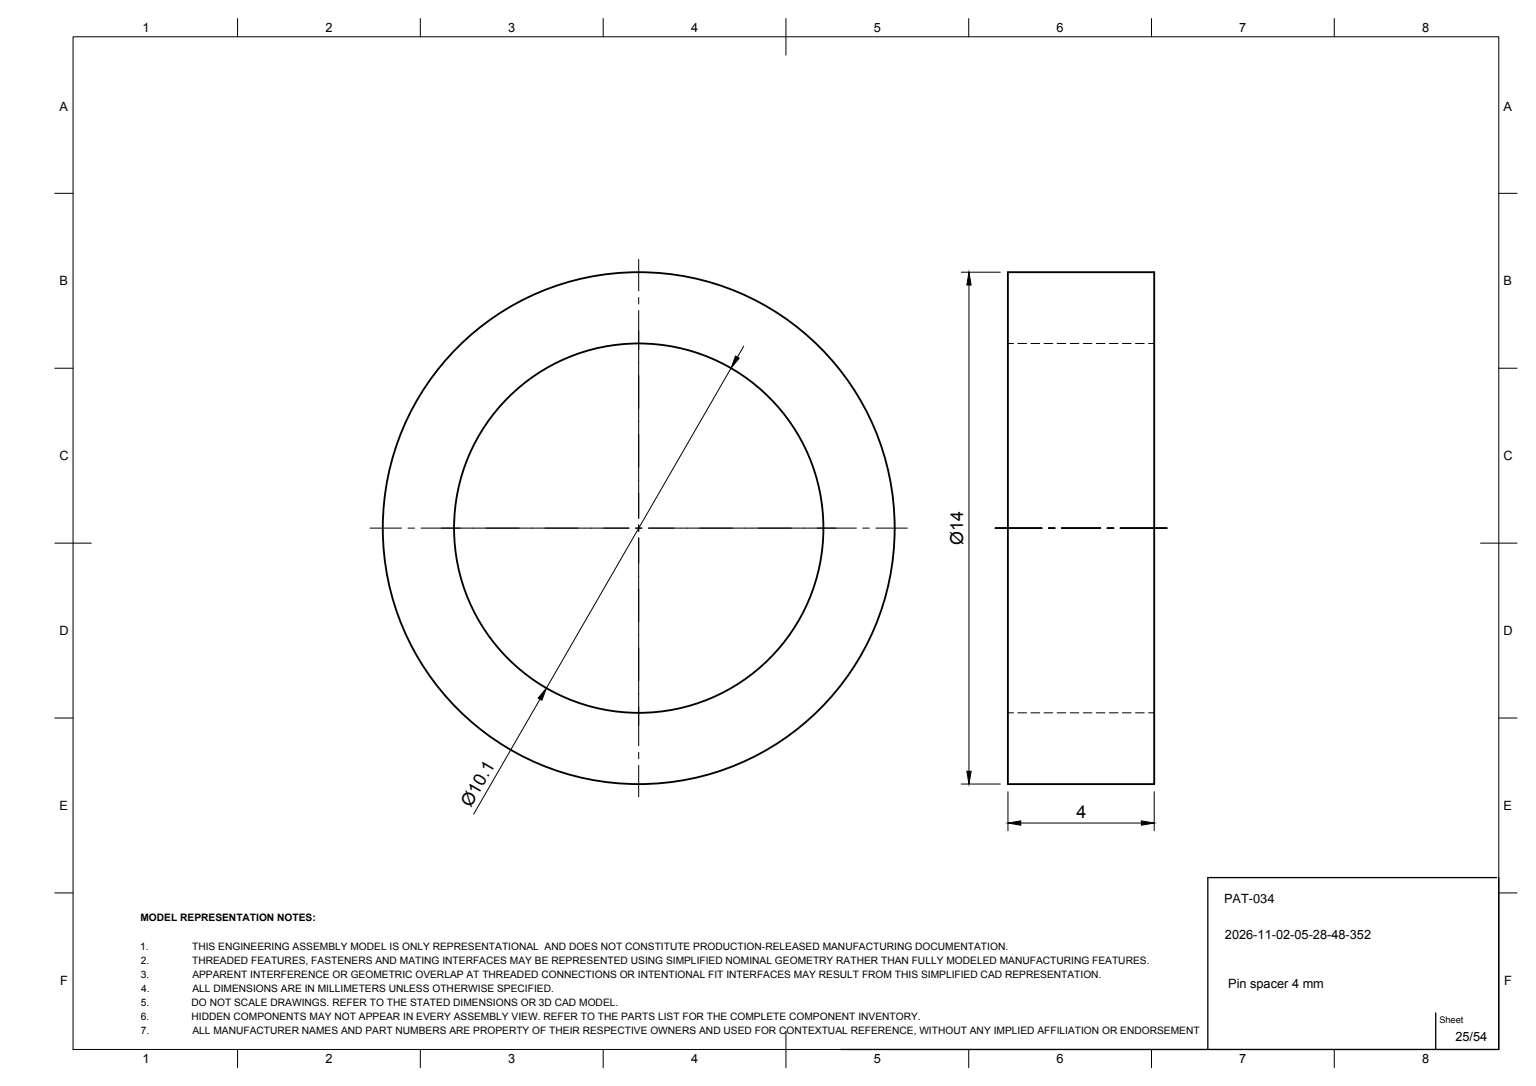
ISO-10303-21;
HEADER;
/* Generated by software containing ST-Developer
 * from STEP Tools, Inc. (www.steptools.com) 
 */

FILE_DESCRIPTION(
/* description */ ('Fatigue rig crank-slider'),
/* implementation_level */ '2;1');

FILE_NAME(
/* name */ 'Pin spacer 4 mm.step',
/* time_stamp */ '2026-10-28T03:24:50-07:00',
/* author */ (''),
/* organization */ (''),
/* preprocessor_version */ 'ST-DEVELOPER v20.2',
/* originating_system */ 'Autodesk Translation Framework v15.17.0.0',
/* authorisation */ '');

FILE_SCHEMA (('AUTOMOTIVE_DESIGN { 1 0 10303 214 3 1 1 }'));
ENDSEC;

DATA;
#10=MECHANICAL_DESIGN_GEOMETRIC_PRESENTATION_REPRESENTATION('',(#611),#16911);
#510=SHAPE_REPRESENTATION_RELATIONSHIP('SRR','None',#17151,#560);
#560=ADVANCED_BREP_SHAPE_REPRESENTATION('',(#668),#16880);
#611=STYLED_ITEM('',(#17487),#668);
#668=MANIFOLD_SOLID_BREP('Body1',#8904);
#837=FACE_BOUND('',#2151,.T.);
#838=FACE_BOUND('',#2153,.T.);
#1059=PLANE('',#10013);
#1060=PLANE('',#10014);
#1488=FACE_OUTER_BOUND('',#2148,.T.);
#1489=FACE_OUTER_BOUND('',#2149,.T.);
#1490=FACE_OUTER_BOUND('',#2150,.T.);
#1491=FACE_OUTER_BOUND('',#2152,.T.);
#2148=EDGE_LOOP('',(#7134,#7135,#7136,#7137));
#2149=EDGE_LOOP('',(#7138,#7139,#7140,#7141));
#2150=EDGE_LOOP('',(#7142));
#2151=EDGE_LOOP('',(#7143));
#2152=EDGE_LOOP('',(#7144));
#2153=EDGE_LOOP('',(#7145));
#2780=LINE('',#15198,#3426);
#2781=LINE('',#15204,#3427);
#3426=VECTOR('',#11918,0.505);
#3427=VECTOR('',#11925,0.7);
#3965=CIRCLE('',#10008,0.505);
#3966=CIRCLE('',#10009,0.505);
#3967=CIRCLE('',#10011,0.7);
#3968=CIRCLE('',#10012,0.7);
#4537=VERTEX_POINT('',#15195);
#4538=VERTEX_POINT('',#15197);
#4539=VERTEX_POINT('',#15201);
#4540=VERTEX_POINT('',#15203);
#5465=EDGE_CURVE('',#4537,#4537,#3965,.T.);
#5466=EDGE_CURVE('',#4537,#4538,#2780,.T.);
#5467=EDGE_CURVE('',#4538,#4538,#3966,.T.);
#5468=EDGE_CURVE('',#4539,#4539,#3967,.T.);
#5469=EDGE_CURVE('',#4539,#4540,#2781,.T.);
#5470=EDGE_CURVE('',#4540,#4540,#3968,.T.);
#7134=ORIENTED_EDGE('',*,*,#5465,.F.);
#7135=ORIENTED_EDGE('',*,*,#5466,.T.);
#7136=ORIENTED_EDGE('',*,*,#5467,.T.);
#7137=ORIENTED_EDGE('',*,*,#5466,.F.);
#7138=ORIENTED_EDGE('',*,*,#5468,.F.);
#7139=ORIENTED_EDGE('',*,*,#5469,.T.);
#7140=ORIENTED_EDGE('',*,*,#5470,.T.);
#7141=ORIENTED_EDGE('',*,*,#5469,.F.);
#7142=ORIENTED_EDGE('',*,*,#5468,.T.);
#7143=ORIENTED_EDGE('',*,*,#5465,.T.);
#7144=ORIENTED_EDGE('',*,*,#5470,.F.);
#7145=ORIENTED_EDGE('',*,*,#5467,.F.);
#8296=CYLINDRICAL_SURFACE('',#10007,0.505);
#8297=CYLINDRICAL_SURFACE('',#10010,0.7);
#8626=ADVANCED_FACE('',(#1488),#8296,.F.);
#8627=ADVANCED_FACE('',(#1489),#8297,.T.);
#8628=ADVANCED_FACE('',(#1490,#837),#1059,.T.);
#8629=ADVANCED_FACE('',(#1491,#838),#1060,.F.);
#8904=CLOSED_SHELL('',(#8626,#8627,#8628,#8629));
#10006=AXIS2_PLACEMENT_3D('',#15193,#11912,#11913);
#10007=AXIS2_PLACEMENT_3D('',#15194,#11914,#11915);
#10008=AXIS2_PLACEMENT_3D('',#15196,#11916,#11917);
#10009=AXIS2_PLACEMENT_3D('',#15199,#11919,#11920);
#10010=AXIS2_PLACEMENT_3D('',#15200,#11921,#11922);
#10011=AXIS2_PLACEMENT_3D('',#15202,#11923,#11924);
#10012=AXIS2_PLACEMENT_3D('',#15205,#11926,#11927);
#10013=AXIS2_PLACEMENT_3D('',#15206,#11928,#11929);
#10014=AXIS2_PLACEMENT_3D('',#15207,#11930,#11931);
#11912=DIRECTION('axis',(0.,0.,1.));
#11913=DIRECTION('refdir',(1.,0.,0.));
#11914=DIRECTION('center_axis',(0.,1.,0.));
#11915=DIRECTION('ref_axis',(1.,0.,0.));
#11916=DIRECTION('center_axis',(0.,-1.,0.));
#11917=DIRECTION('ref_axis',(1.,0.,0.));
#11918=DIRECTION('',(0.,-1.,0.));
#11919=DIRECTION('center_axis',(0.,-1.,0.));
#11920=DIRECTION('ref_axis',(1.,0.,0.));
#11921=DIRECTION('center_axis',(0.,1.,0.));
#11922=DIRECTION('ref_axis',(1.,0.,0.));
#11923=DIRECTION('center_axis',(0.,1.,0.));
#11924=DIRECTION('ref_axis',(1.,0.,0.));
#11925=DIRECTION('',(0.,-1.,0.));
#11926=DIRECTION('center_axis',(0.,1.,0.));
#11927=DIRECTION('ref_axis',(1.,0.,0.));
#11928=DIRECTION('center_axis',(0.,1.,0.));
#11929=DIRECTION('ref_axis',(1.,0.,0.));
#11930=DIRECTION('center_axis',(0.,1.,0.));
#11931=DIRECTION('ref_axis',(1.,0.,0.));
#15193=CARTESIAN_POINT('',(0.,0.,0.));
#15194=CARTESIAN_POINT('Origin',(1.,4.4,12.));
#15195=CARTESIAN_POINT('',(0.495,4.8,12.));
#15196=CARTESIAN_POINT('Origin',(1.,4.8,12.));
#15197=CARTESIAN_POINT('',(0.495,4.4,12.));
#15198=CARTESIAN_POINT('',(0.495,4.4,12.));
#15199=CARTESIAN_POINT('Origin',(1.,4.4,12.));
#15200=CARTESIAN_POINT('Origin',(1.,4.4,12.));
#15201=CARTESIAN_POINT('',(0.3,4.8,12.));
#15202=CARTESIAN_POINT('Origin',(1.,4.8,12.));
#15203=CARTESIAN_POINT('',(0.3,4.4,12.));
#15204=CARTESIAN_POINT('',(0.3,4.4,12.));
#15205=CARTESIAN_POINT('Origin',(1.,4.4,12.));
#15206=CARTESIAN_POINT('Origin',(1.,4.8,12.));
#15207=CARTESIAN_POINT('Origin',(1.,4.4,12.));
#16821=UNCERTAINTY_MEASURE_WITH_UNIT(LENGTH_MEASURE(0.001),#16912,
'DISTANCE_ACCURACY_VALUE',
'Maximum model space distance between geometric entities at asserted c
onnectivities');
#16852=UNCERTAINTY_MEASURE_WITH_UNIT(LENGTH_MEASURE(0.001),#16912,
'DISTANCE_ACCURACY_VALUE',
'Maximum model space distance between geometric entities at asserted c
onnectivities');
#16880=(
GEOMETRIC_REPRESENTATION_CONTEXT(3)
GLOBAL_UNCERTAINTY_ASSIGNED_CONTEXT((#16821))
GLOBAL_UNIT_ASSIGNED_CONTEXT((#16912,#16914,#16915))
REPRESENTATION_CONTEXT('','3D')
);
#16911=(
GEOMETRIC_REPRESENTATION_CONTEXT(3)
GLOBAL_UNCERTAINTY_ASSIGNED_CONTEXT((#16852))
GLOBAL_UNIT_ASSIGNED_CONTEXT((#16912,#16914,#16915))
REPRESENTATION_CONTEXT('','3D')
);
#16912=(
LENGTH_UNIT()
NAMED_UNIT(*)
SI_UNIT(.CENTI.,.METRE.)
);
#16914=(
NAMED_UNIT(*)
PLANE_ANGLE_UNIT()
SI_UNIT($,.RADIAN.)
);
#16915=(
NAMED_UNIT(*)
SI_UNIT($,.STERADIAN.)
SOLID_ANGLE_UNIT()
);
#16943=SHAPE_DEFINITION_REPRESENTATION(#17003,#17151);
#17003=PRODUCT_DEFINITION_SHAPE('',$,#17210);
#17151=SHAPE_REPRESENTATION('',(#10006),#16880);
#17182=PRODUCT_DEFINITION_CONTEXT('part definition',#17358,'design');
#17210=PRODUCT_DEFINITION('Pin spacer 4 mm','Pin spacer 4 mm',#17268,#17182);
#17268=PRODUCT_DEFINITION_FORMATION('',$,#17387);
#17358=APPLICATION_CONTEXT(
'Core Data for Automotive Mechanical Design Process');
#17359=PRODUCT_CONTEXT('part definition',#17358,'mechanical');
#17387=PRODUCT('Pin spacer 4 mm','Pin spacer 4 mm','Pin spacer 4 mm',(#17359));
#17481=COLOUR_RGB('Grey',0.48,0.52,0.57);
#17482=FILL_AREA_STYLE_COLOUR('',#17481);
#17483=FILL_AREA_STYLE('',(#17482));
#17484=SURFACE_STYLE_FILL_AREA(#17483);
#17485=SURFACE_SIDE_STYLE('',(#17484));
#17486=SURFACE_STYLE_USAGE(.BOTH.,#17485);
#17487=PRESENTATION_STYLE_ASSIGNMENT((#17486));
ENDSEC;
END-ISO-10303-21;
